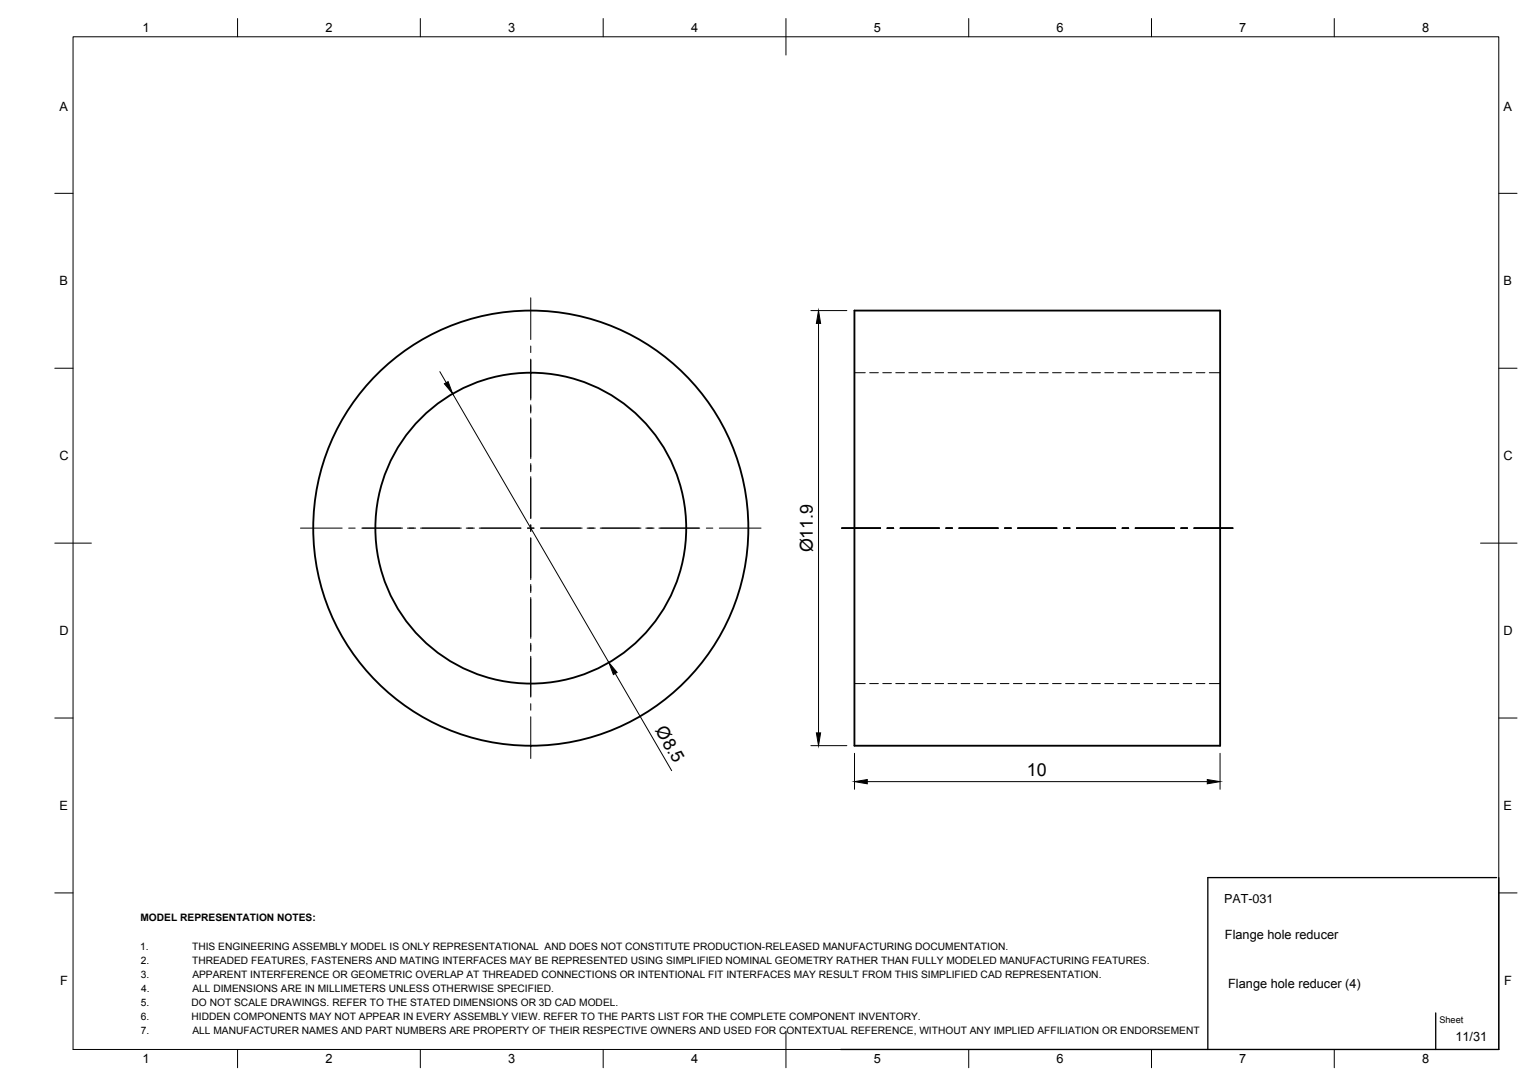
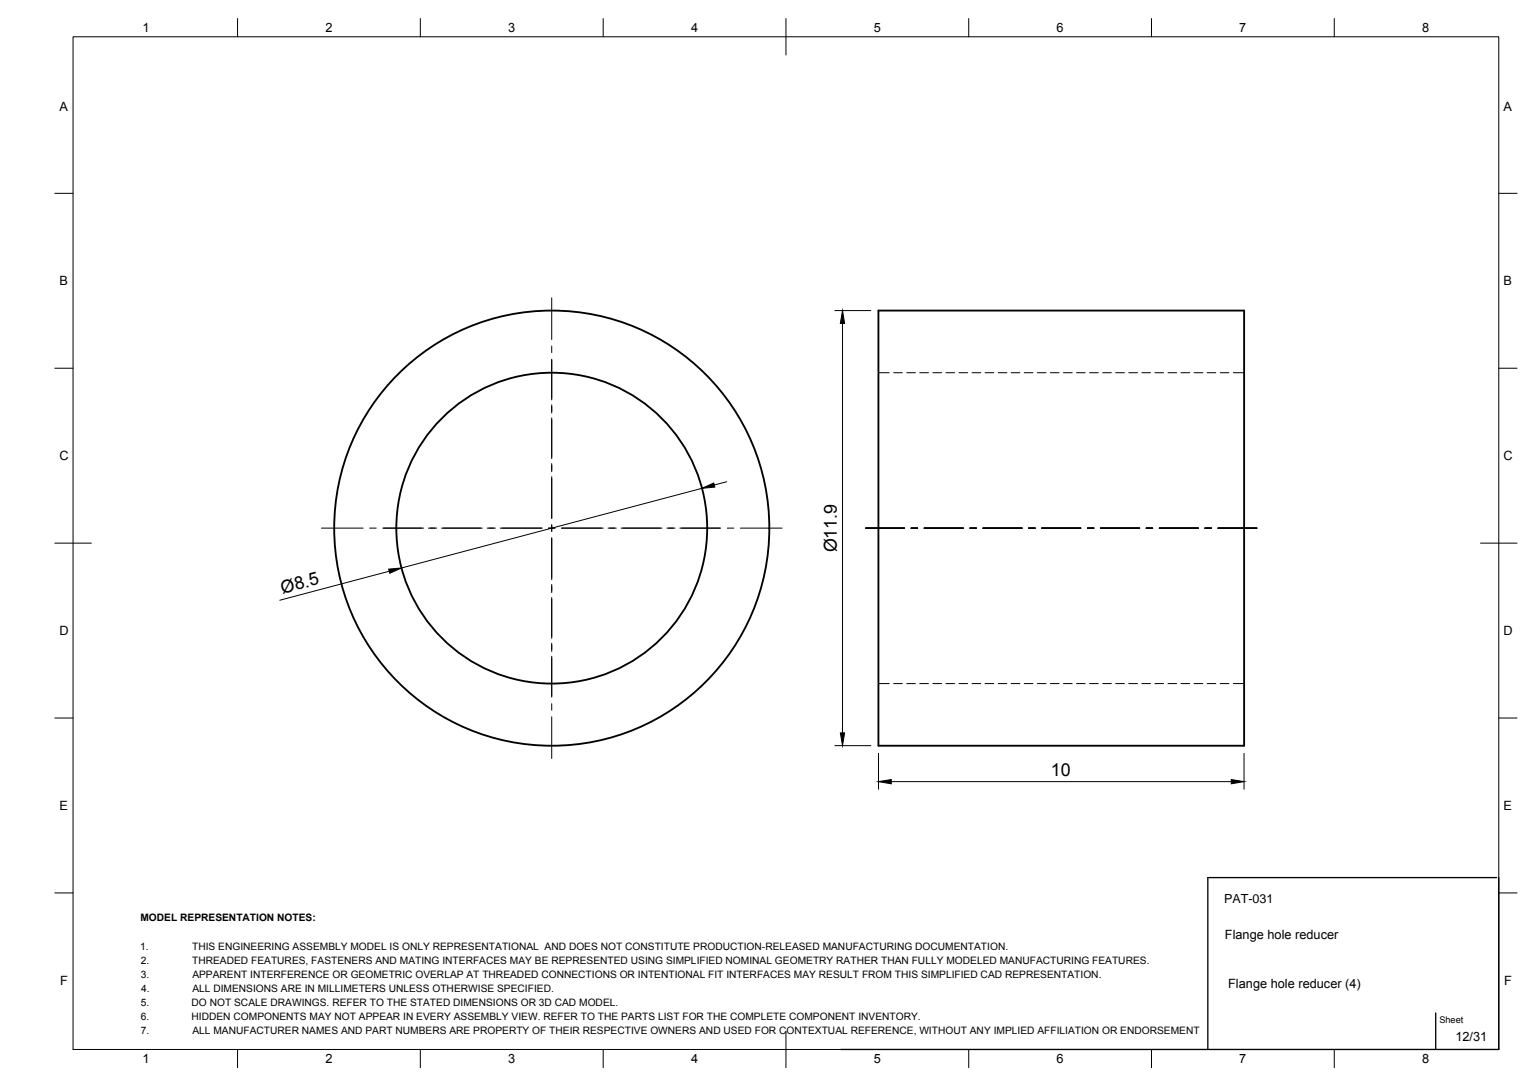
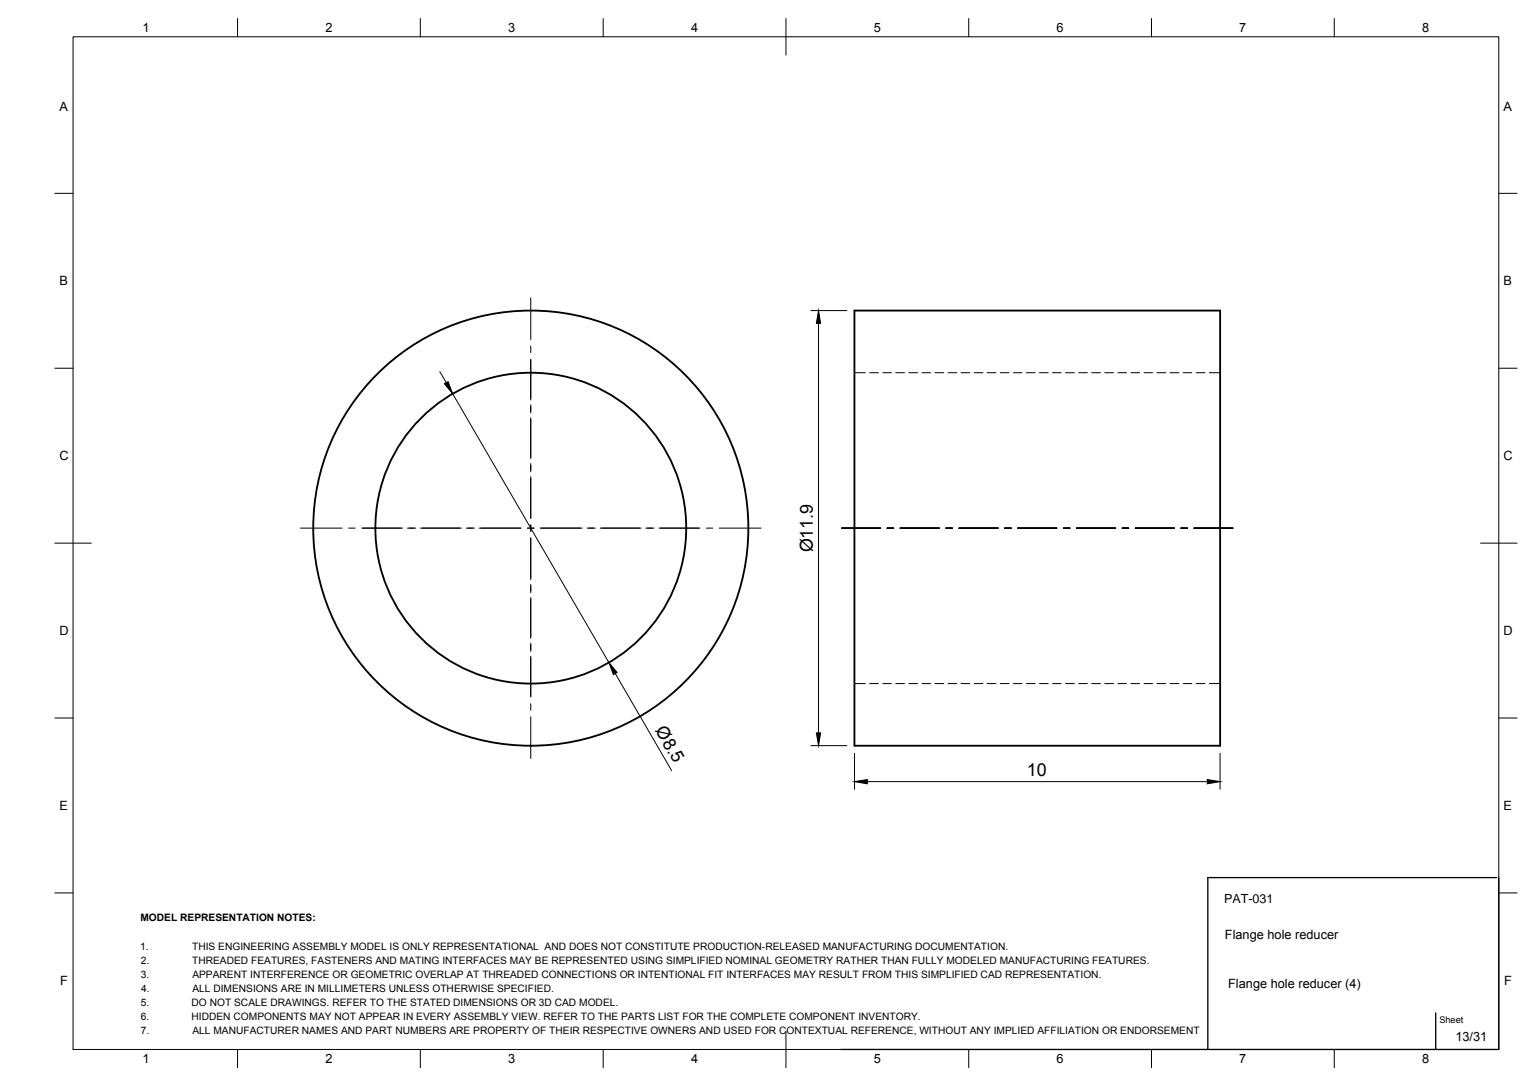
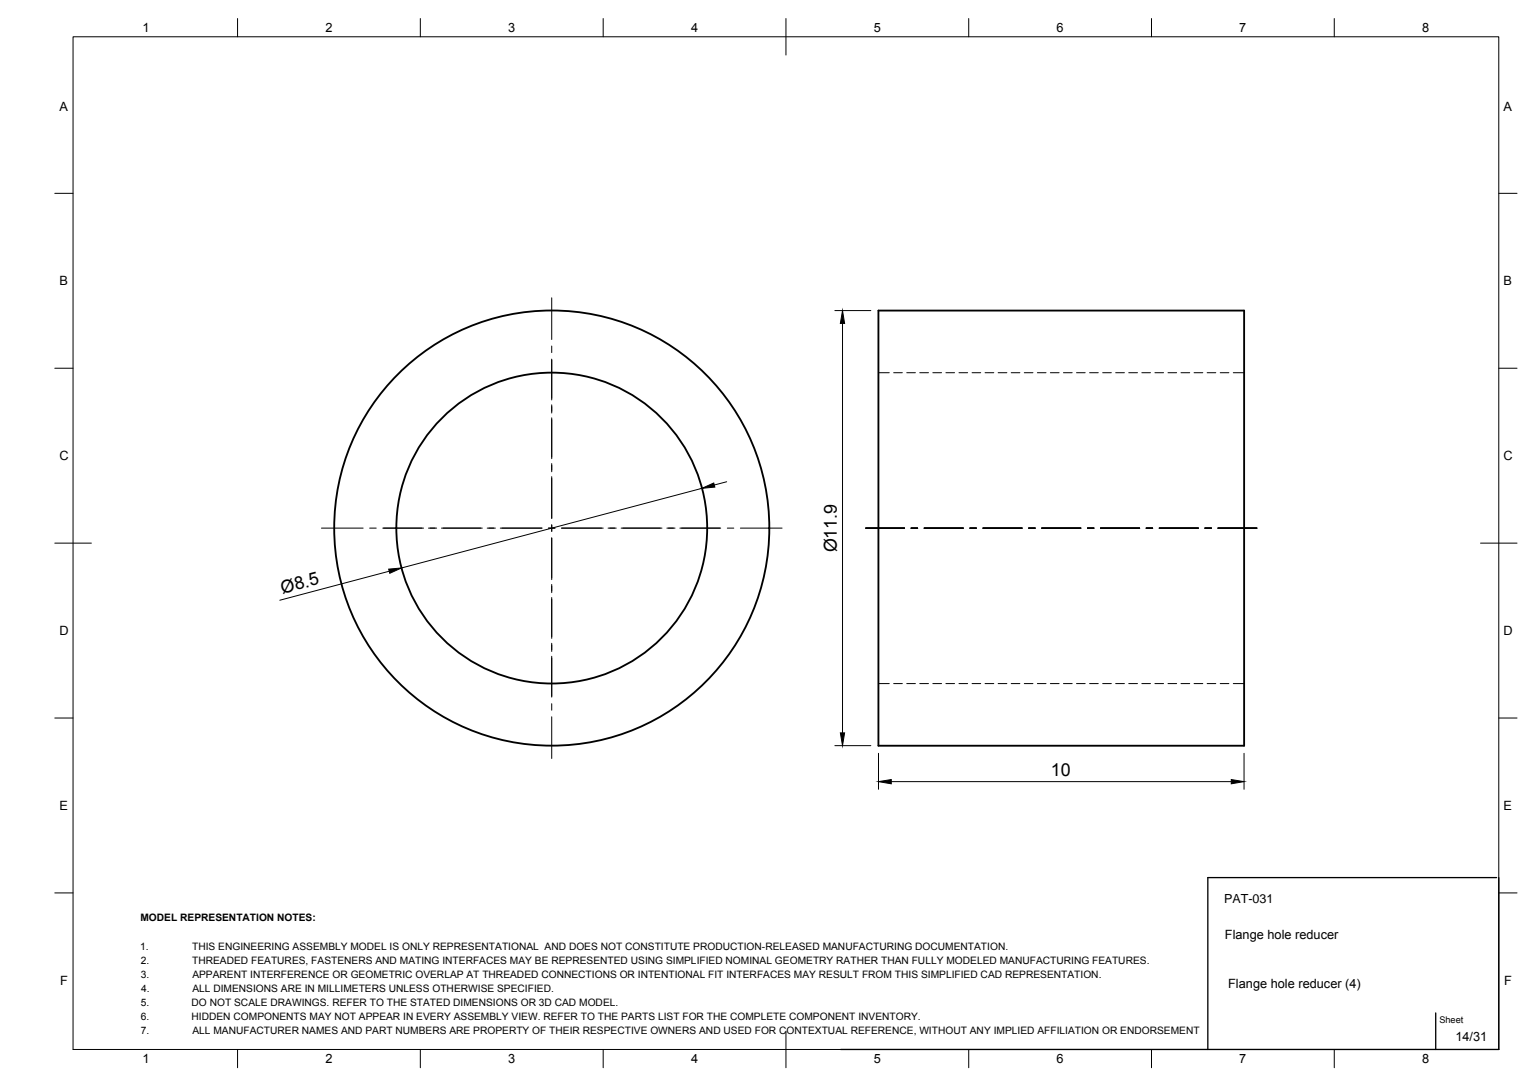
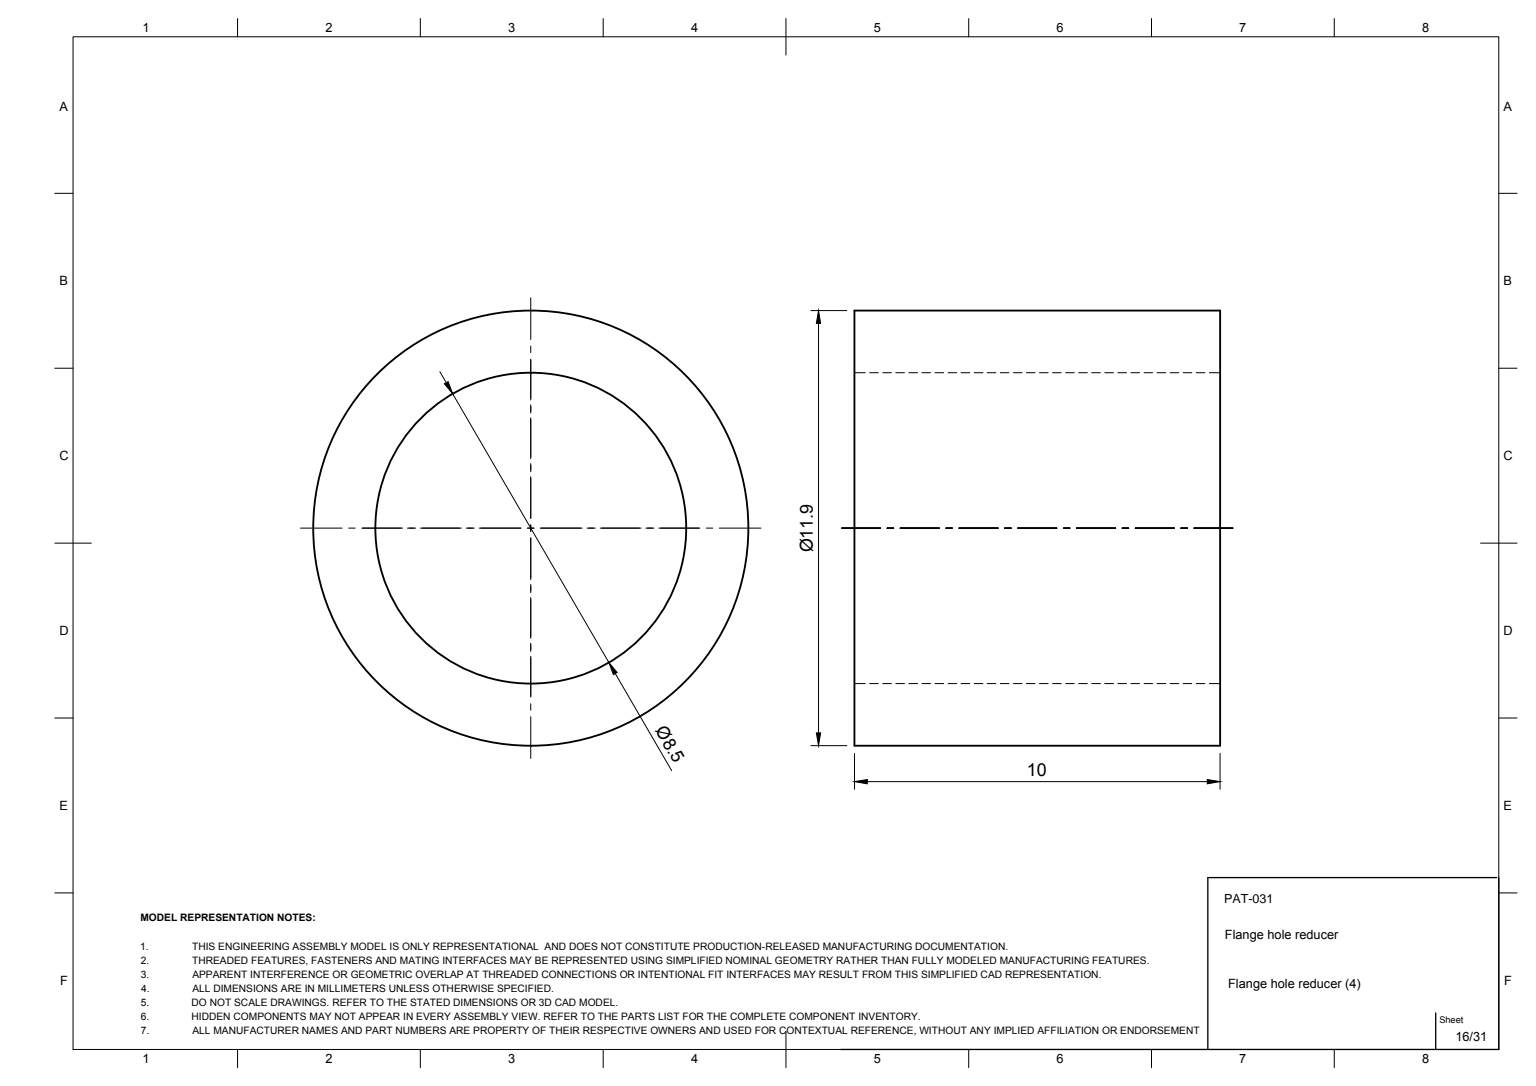
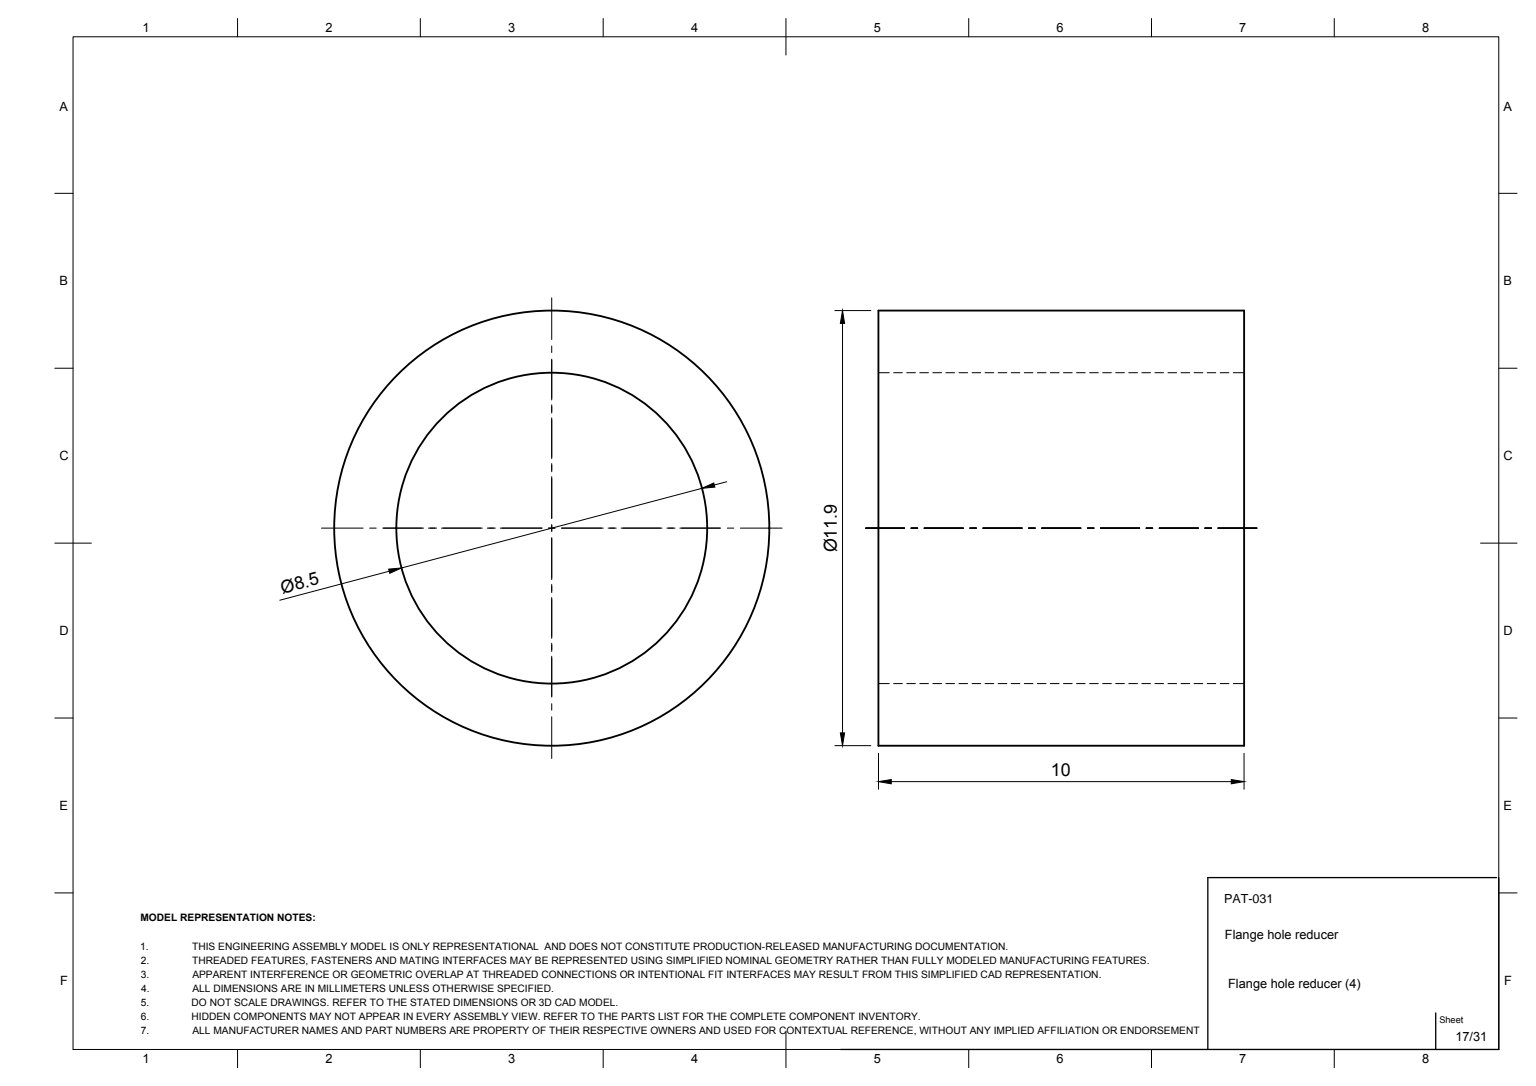
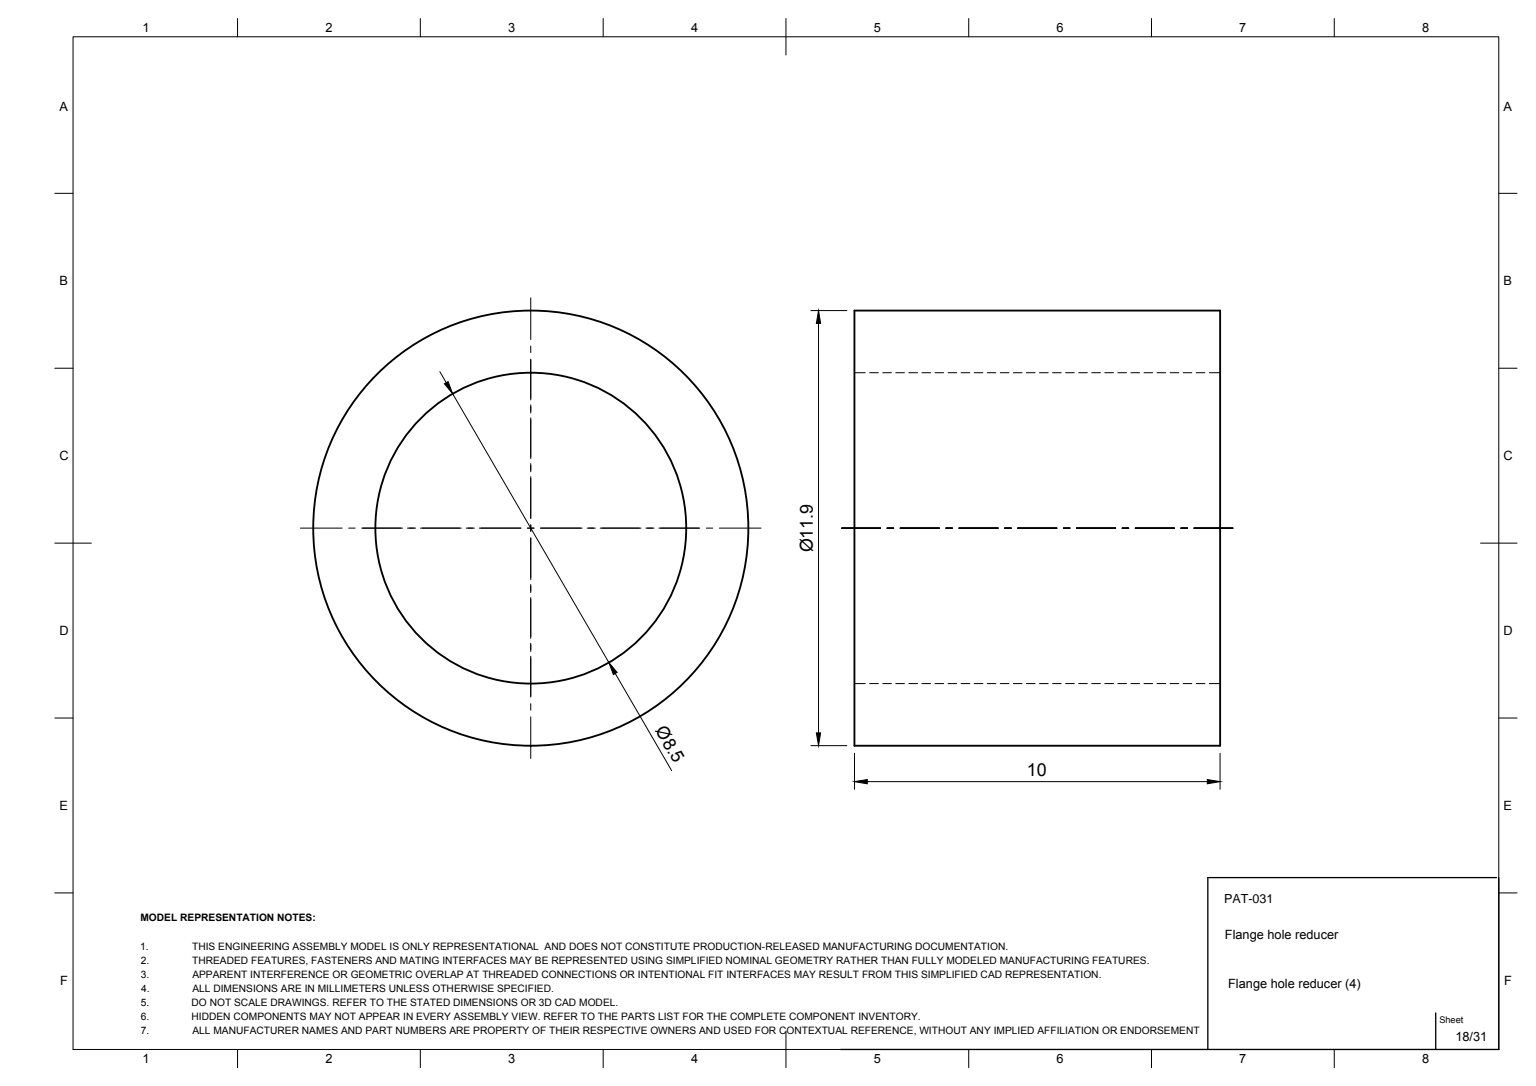
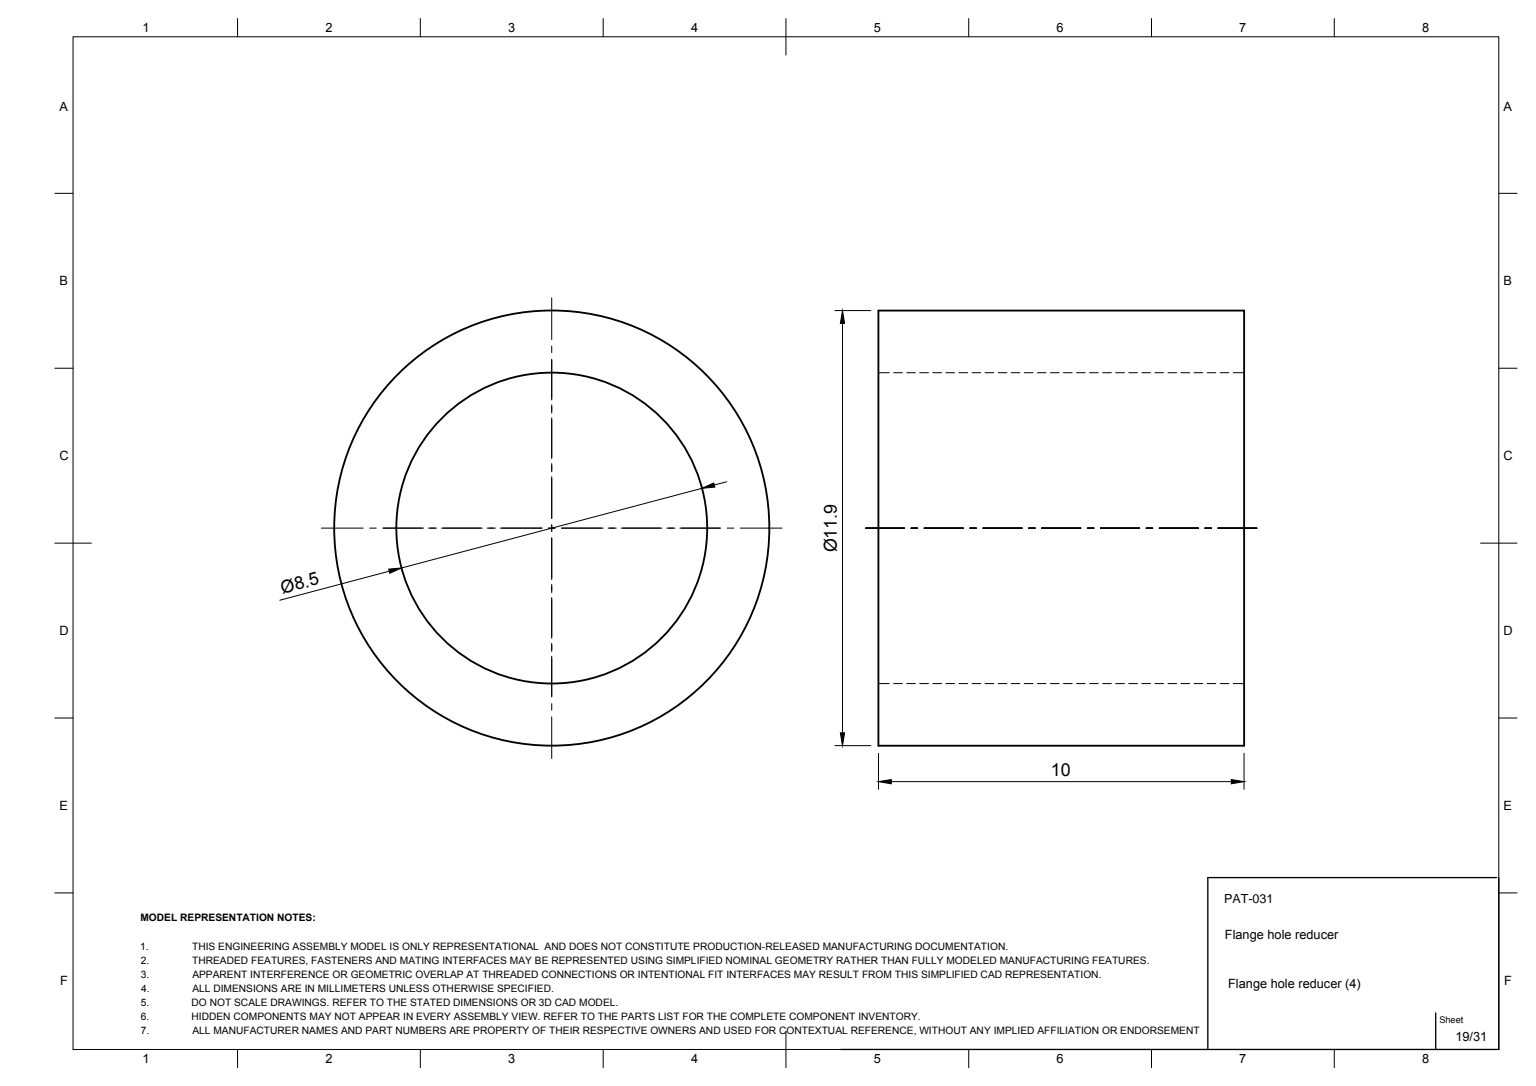
ISO-10303-21;
HEADER;
/* Generated by software containing ST-Developer
 * from STEP Tools, Inc. (www.steptools.com) 
 */

FILE_DESCRIPTION(
/* description */ ('Double-row support with tensioned shaft'),
/* implementation_level */ '2;1');

FILE_NAME(
/* name */ 'Flange hole reducer.step',
/* time_stamp */ '2026-10-27T10:50:35-07:00',
/* author */ (''),
/* organization */ (''),
/* preprocessor_version */ 'ST-DEVELOPER v20.2',
/* originating_system */ 'Autodesk Translation Framework v15.17.0.0',
/* authorisation */ '');

FILE_SCHEMA (('AUTOMOTIVE_DESIGN { 1 0 10303 214 3 1 1 }'));
ENDSEC;

DATA;
#10=MECHANICAL_DESIGN_GEOMETRIC_PRESENTATION_REPRESENTATION('',(#485),#11559);
#421=SHAPE_REPRESENTATION_RELATIONSHIP('SRR','None',#11729,#453);
#453=ADVANCED_BREP_SHAPE_REPRESENTATION('',(#518),#11531);
#485=STYLED_ITEM('',(#11981),#518);
#518=MANIFOLD_SOLID_BREP('Body1',#6330);
#580=FACE_BOUND('',#1359,.T.);
#581=FACE_BOUND('',#1361,.T.);
#717=PLANE('',#6823);
#718=PLANE('',#6824);
#974=FACE_OUTER_BOUND('',#1356,.T.);
#975=FACE_OUTER_BOUND('',#1357,.T.);
#976=FACE_OUTER_BOUND('',#1358,.T.);
#977=FACE_OUTER_BOUND('',#1360,.T.);
#1356=EDGE_LOOP('',(#4600,#4601,#4602,#4603));
#1357=EDGE_LOOP('',(#4604,#4605,#4606,#4607));
#1358=EDGE_LOOP('',(#4608));
#1359=EDGE_LOOP('',(#4609));
#1360=EDGE_LOOP('',(#4610));
#1361=EDGE_LOOP('',(#4611));
#1839=LINE('',#9529,#2386);
#1840=LINE('',#9535,#2387);
#2386=VECTOR('',#7680,0.425);
#2387=VECTOR('',#7687,0.595);
#2874=CIRCLE('',#6818,0.425);
#2875=CIRCLE('',#6819,0.425);
#2876=CIRCLE('',#6821,0.595);
#2877=CIRCLE('',#6822,0.595);
#3117=VERTEX_POINT('',#9526);
#3118=VERTEX_POINT('',#9528);
#3119=VERTEX_POINT('',#9532);
#3120=VERTEX_POINT('',#9534);
#3685=EDGE_CURVE('',#3117,#3117,#2874,.T.);
#3686=EDGE_CURVE('',#3117,#3118,#1839,.T.);
#3687=EDGE_CURVE('',#3118,#3118,#2875,.T.);
#3688=EDGE_CURVE('',#3119,#3119,#2876,.T.);
#3689=EDGE_CURVE('',#3119,#3120,#1840,.T.);
#3690=EDGE_CURVE('',#3120,#3120,#2877,.T.);
#4600=ORIENTED_EDGE('',*,*,#3685,.F.);
#4601=ORIENTED_EDGE('',*,*,#3686,.T.);
#4602=ORIENTED_EDGE('',*,*,#3687,.T.);
#4603=ORIENTED_EDGE('',*,*,#3686,.F.);
#4604=ORIENTED_EDGE('',*,*,#3688,.F.);
#4605=ORIENTED_EDGE('',*,*,#3689,.T.);
#4606=ORIENTED_EDGE('',*,*,#3690,.T.);
#4607=ORIENTED_EDGE('',*,*,#3689,.F.);
#4608=ORIENTED_EDGE('',*,*,#3688,.T.);
#4609=ORIENTED_EDGE('',*,*,#3685,.T.);
#4610=ORIENTED_EDGE('',*,*,#3690,.F.);
#4611=ORIENTED_EDGE('',*,*,#3687,.F.);
#5909=CYLINDRICAL_SURFACE('',#6817,0.425);
#5910=CYLINDRICAL_SURFACE('',#6820,0.595);
#6037=ADVANCED_FACE('',(#974),#5909,.F.);
#6038=ADVANCED_FACE('',(#975),#5910,.T.);
#6039=ADVANCED_FACE('',(#976,#580),#717,.T.);
#6040=ADVANCED_FACE('',(#977,#581),#718,.F.);
#6330=CLOSED_SHELL('',(#6037,#6038,#6039,#6040));
#6816=AXIS2_PLACEMENT_3D('',#9524,#7674,#7675);
#6817=AXIS2_PLACEMENT_3D('',#9525,#7676,#7677);
#6818=AXIS2_PLACEMENT_3D('',#9527,#7678,#7679);
#6819=AXIS2_PLACEMENT_3D('',#9530,#7681,#7682);
#6820=AXIS2_PLACEMENT_3D('',#9531,#7683,#7684);
#6821=AXIS2_PLACEMENT_3D('',#9533,#7685,#7686);
#6822=AXIS2_PLACEMENT_3D('',#9536,#7688,#7689);
#6823=AXIS2_PLACEMENT_3D('',#9537,#7690,#7691);
#6824=AXIS2_PLACEMENT_3D('',#9538,#7692,#7693);
#7674=DIRECTION('axis',(0.,0.,1.));
#7675=DIRECTION('refdir',(1.,0.,0.));
#7676=DIRECTION('center_axis',(0.,1.,0.));
#7677=DIRECTION('ref_axis',(1.,0.,0.));
#7678=DIRECTION('center_axis',(0.,-1.,0.));
#7679=DIRECTION('ref_axis',(1.,0.,0.));
#7680=DIRECTION('',(0.,-1.,0.));
#7681=DIRECTION('center_axis',(0.,-1.,0.));
#7682=DIRECTION('ref_axis',(1.,0.,0.));
#7683=DIRECTION('center_axis',(0.,1.,0.));
#7684=DIRECTION('ref_axis',(1.,0.,0.));
#7685=DIRECTION('center_axis',(0.,1.,0.));
#7686=DIRECTION('ref_axis',(1.,0.,0.));
#7687=DIRECTION('',(0.,-1.,0.));
#7688=DIRECTION('center_axis',(0.,1.,0.));
#7689=DIRECTION('ref_axis',(1.,0.,0.));
#7690=DIRECTION('center_axis',(0.,1.,0.));
#7691=DIRECTION('ref_axis',(1.,0.,0.));
#7692=DIRECTION('center_axis',(0.,1.,0.));
#7693=DIRECTION('ref_axis',(1.,0.,0.));
#9524=CARTESIAN_POINT('',(0.,0.,0.));
#9525=CARTESIAN_POINT('Origin',(-3.2,-0.5,6.8));
#9526=CARTESIAN_POINT('',(-3.625,0.5,6.8));
#9527=CARTESIAN_POINT('Origin',(-3.2,0.5,6.8));
#9528=CARTESIAN_POINT('',(-3.625,-0.5,6.8));
#9529=CARTESIAN_POINT('',(-3.625,-0.5,6.8));
#9530=CARTESIAN_POINT('Origin',(-3.2,-0.5,6.8));
#9531=CARTESIAN_POINT('Origin',(-3.2,-0.5,6.8));
#9532=CARTESIAN_POINT('',(-3.795,0.5,6.8));
#9533=CARTESIAN_POINT('Origin',(-3.2,0.5,6.8));
#9534=CARTESIAN_POINT('',(-3.795,-0.5,6.8));
#9535=CARTESIAN_POINT('',(-3.795,-0.5,6.8));
#9536=CARTESIAN_POINT('Origin',(-3.2,-0.5,6.8));
#9537=CARTESIAN_POINT('Origin',(-3.2,0.5,6.8));
#9538=CARTESIAN_POINT('Origin',(-3.2,-0.5,6.8));
#11494=UNCERTAINTY_MEASURE_WITH_UNIT(LENGTH_MEASURE(0.001),#11560,
'DISTANCE_ACCURACY_VALUE',
'Maximum model space distance between geometric entities at asserted c
onnectivities');
#11522=UNCERTAINTY_MEASURE_WITH_UNIT(LENGTH_MEASURE(0.001),#11560,
'DISTANCE_ACCURACY_VALUE',
'Maximum model space distance between geometric entities at asserted c
onnectivities');
#11531=(
GEOMETRIC_REPRESENTATION_CONTEXT(3)
GLOBAL_UNCERTAINTY_ASSIGNED_CONTEXT((#11494))
GLOBAL_UNIT_ASSIGNED_CONTEXT((#11560,#11562,#11563))
REPRESENTATION_CONTEXT('','3D')
);
#11559=(
GEOMETRIC_REPRESENTATION_CONTEXT(3)
GLOBAL_UNCERTAINTY_ASSIGNED_CONTEXT((#11522))
GLOBAL_UNIT_ASSIGNED_CONTEXT((#11560,#11562,#11563))
REPRESENTATION_CONTEXT('','3D')
);
#11560=(
LENGTH_UNIT()
NAMED_UNIT(*)
SI_UNIT(.CENTI.,.METRE.)
);
#11562=(
NAMED_UNIT(*)
PLANE_ANGLE_UNIT()
SI_UNIT($,.RADIAN.)
);
#11563=(
NAMED_UNIT(*)
SI_UNIT($,.STERADIAN.)
SOLID_ANGLE_UNIT()
);
#11572=SHAPE_DEFINITION_REPRESENTATION(#11608,#11729);
#11608=PRODUCT_DEFINITION_SHAPE('',$,#11766);
#11729=SHAPE_REPRESENTATION('',(#6816),#11531);
#11757=PRODUCT_DEFINITION_CONTEXT('part definition',#11867,'design');
#11766=PRODUCT_DEFINITION('Flange hole reducer','Flange hole reducer',#11802,
#11757);
#11802=PRODUCT_DEFINITION_FORMATION('',$,#11877);
#11867=APPLICATION_CONTEXT(
'Core Data for Automotive Mechanical Design Process');
#11868=PRODUCT_CONTEXT('part definition',#11867,'mechanical');
#11877=PRODUCT('Flange hole reducer','Flange hole reducer',
'Flange hole reducer',(#11868));
#11975=COLOUR_RGB('Off White',0.89,0.88,0.83);
#11976=FILL_AREA_STYLE_COLOUR('',#11975);
#11977=FILL_AREA_STYLE('',(#11976));
#11978=SURFACE_STYLE_FILL_AREA(#11977);
#11979=SURFACE_SIDE_STYLE('',(#11978));
#11980=SURFACE_STYLE_USAGE(.BOTH.,#11979);
#11981=PRESENTATION_STYLE_ASSIGNMENT((#11980));
ENDSEC;
END-ISO-10303-21;
